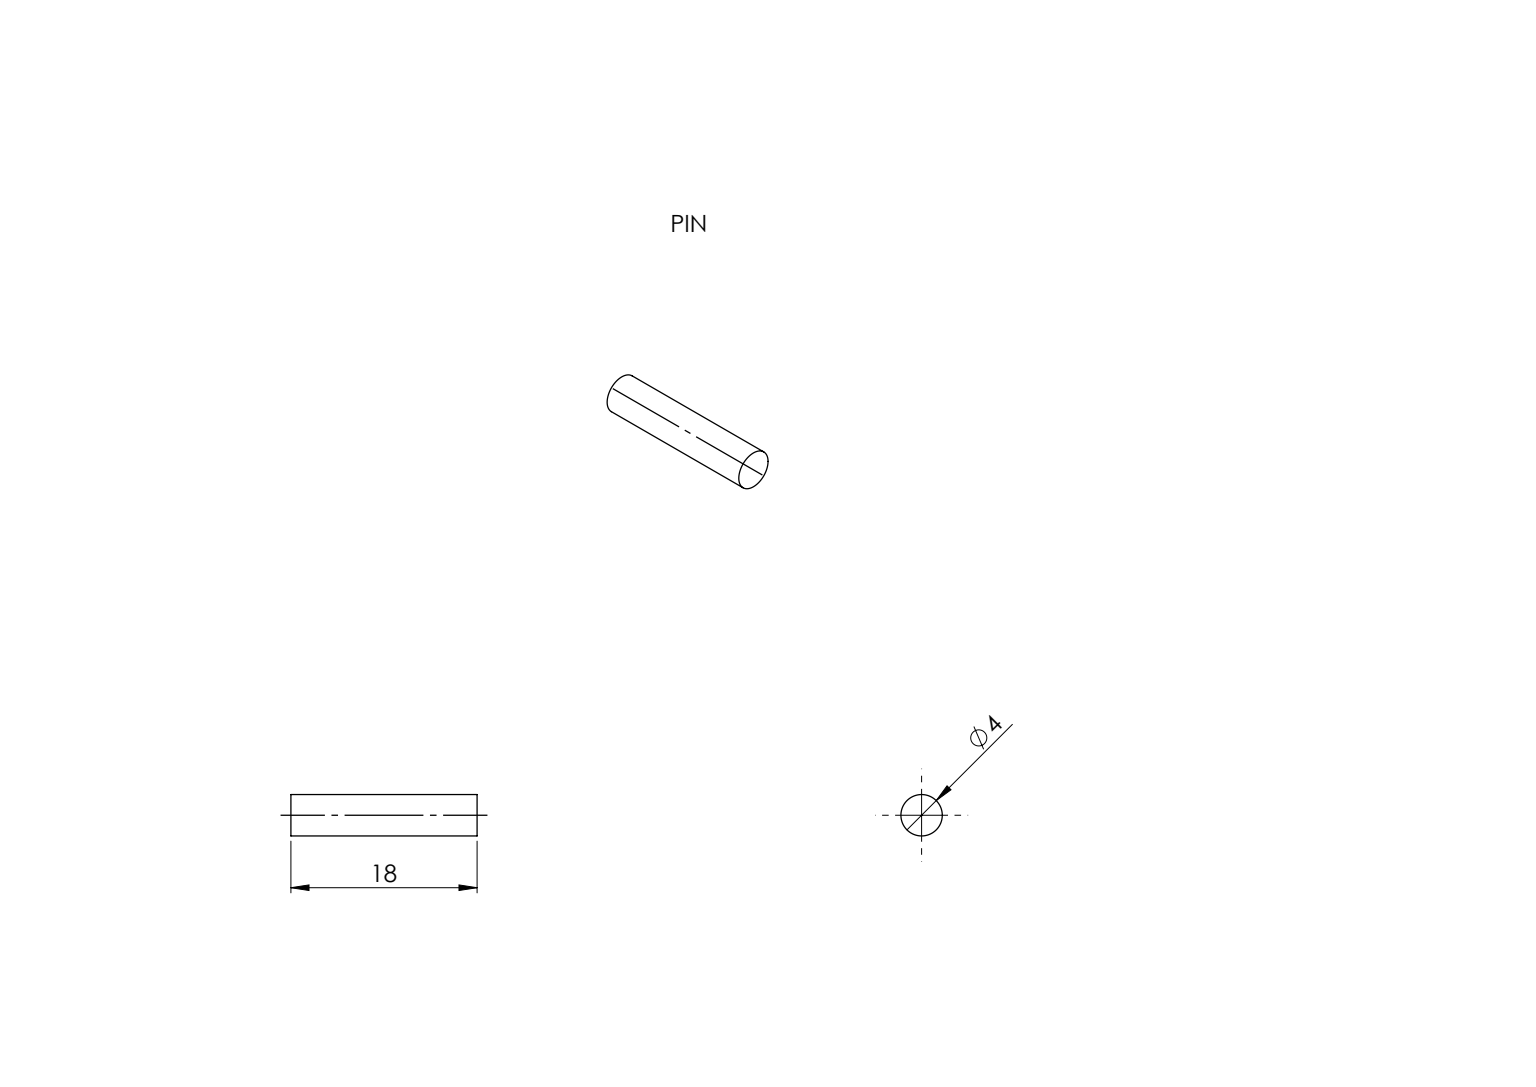
ISO-10303-21;
HEADER;
FILE_DESCRIPTION (('STEP AP214'),
    '1' );
FILE_NAME ('pin.step',
    '2026-10-03T18:28:46',
    ( '' ),
    ( '' ),
    'SwSTEP 2.0',
    'SolidWorks 2026',
    '' );
FILE_SCHEMA (( 'AUTOMOTIVE_DESIGN' ));
ENDSEC;

DATA;
#1=( LENGTH_UNIT ( ) NAMED_UNIT ( * ) SI_UNIT ( .MILLI., .METRE. ) );
#130=DIRECTION ( 'NONE',  ( 0.000000000000000000, 0.000000000000000000, -1.000000000000000000 ) ) ;
#220=ORIENTED_EDGE ( 'NONE', *, *, #9750, .F. ) ;
#239=CARTESIAN_POINT ( 'NONE',  ( 9.000000000000000000, 19.99999999999999645, 13.00000000000000000 ) ) ;
#291=DIRECTION ( 'NONE',  ( -1.000000000000000000, -0.000000000000000000, -0.000000000000000000 ) ) ;
#502=DIRECTION ( 'NONE',  ( 0.000000000000000000, 0.000000000000000000, 1.000000000000000000 ) ) ;
#644=SHAPE_DEFINITION_REPRESENTATION ( #7147, #9430 ) ;
#749=FACE_OUTER_BOUND ( 'NONE', #2071, .T. ) ;
#998=PRESENTATION_STYLE_ASSIGNMENT (( #4868 ) ) ;
#1023=ADVANCED_FACE ( 'NONE', ( #9629 ), #8663, .T. ) ;
#1105=ORIENTED_EDGE ( 'NONE', *, *, #3056, .F. ) ;
#1118=EDGE_CURVE ( 'NONE', #8741, #1470, #4721, .T. ) ;
#1207=ORIENTED_EDGE ( 'NONE', *, *, #4683, .F. ) ;
#1223=EDGE_CURVE ( 'NONE', #9435, #3589, #5730, .T. ) ;
#1293=DIRECTION ( 'NONE',  ( 1.000000000000000000, 0.000000000000000000, 0.000000000000000000 ) ) ;
#1299=CARTESIAN_POINT ( 'NONE',  ( 9.000000000000000000, 19.99999999999999645, 15.00000000000000000 ) ) ;
#1315=FACE_OUTER_BOUND ( 'NONE', #6062, .T. ) ;
#1470=VERTEX_POINT ( 'NONE', #5190 ) ;
#1784=( LENGTH_UNIT ( ) NAMED_UNIT ( * ) SI_UNIT ( .MILLI., .METRE. ) );
#2036=DIRECTION ( 'NONE',  ( 1.000000000000000000, 0.000000000000000000, 0.000000000000000000 ) ) ;
#2057=VECTOR ( 'NONE', #4305, 1000.000000000000000 ) ;
#2071=EDGE_LOOP ( 'NONE', ( #220, #10334, #2999, #7018 ) ) ;
#2090=DIRECTION ( 'NONE',  ( 0.000000000000000000, 0.000000000000000000, -1.000000000000000000 ) ) ;
#2101=AXIS2_PLACEMENT_3D ( 'NONE', #7090, #5610, #4547 ) ;
#2267=( GEOMETRIC_REPRESENTATION_CONTEXT ( 3 ) GLOBAL_UNCERTAINTY_ASSIGNED_CONTEXT ( ( #4377 ) ) GLOBAL_UNIT_ASSIGNED_CONTEXT ( ( #8113, #4925, #8273 ) ) REPRESENTATION_CONTEXT ( 'NONE', 'WORKASPACE' ) );
#2285=DIRECTION ( 'NONE',  ( -1.000000000000000000, -0.000000000000000000, -0.000000000000000000 ) ) ;
#2415=PRODUCT_DEFINITION_CONTEXT ( 'detailed design', #3097, 'design' ) ;
#2443=FILL_AREA_STYLE_COLOUR ( '', #7171 ) ;
#2493=FILL_AREA_STYLE ('',( #2443 ) ) ;
#2596=ADVANCED_FACE ( 'NONE', ( #8570 ), #2893, .T. ) ;
#2877=EDGE_CURVE ( 'NONE', #9435, #1470, #9790, .T. ) ;
#2893=CYLINDRICAL_SURFACE ( 'NONE', #5265, 2.000000000000001776 ) ;
#2947=( GEOMETRIC_REPRESENTATION_CONTEXT ( 3 ) GLOBAL_UNCERTAINTY_ASSIGNED_CONTEXT ( ( #3643 ) ) GLOBAL_UNIT_ASSIGNED_CONTEXT ( ( #1, #6456, #4125 ) ) REPRESENTATION_CONTEXT ( 'NONE', 'WORKASPACE' ) );
#2999=ORIENTED_EDGE ( 'NONE', *, *, #2877, .T. ) ;
#3056=EDGE_CURVE ( 'NONE', #3589, #9435, #8569, .T. ) ;
#3097=APPLICATION_CONTEXT ( 'automotive_design' ) ;
#3267=( NAMED_UNIT ( * ) PLANE_ANGLE_UNIT ( ) SI_UNIT ( $, .RADIAN. ) );
#3270=PRODUCT ( 'pin', 'pin', '', ( #8078 ) ) ;
#3440=ORIENTED_EDGE ( 'NONE', *, *, #2877, .F. ) ;
#3589=VERTEX_POINT ( 'NONE', #8495 ) ;
#3643=UNCERTAINTY_MEASURE_WITH_UNIT (LENGTH_MEASURE( 1.000000000000000082E-05 ), #1, 'distance_accuracy_value', 'NONE');
#3713=AXIS2_PLACEMENT_3D ( 'NONE', #4594, #5496, #7837 ) ;
#3716=ADVANCED_FACE ( 'NONE', ( #749 ), #8594, .T. ) ;
#3808=PRODUCT_DEFINITION_FORMATION_WITH_SPECIFIED_SOURCE ( 'ANY', '', #3270, .NOT_KNOWN. ) ;
#3845=FILL_AREA_STYLE_COLOUR ( '', #6596 ) ;
#4001=AXIS2_PLACEMENT_3D ( 'NONE', #9354, #2036, #2090 ) ;
#4125=( NAMED_UNIT ( * ) SI_UNIT ( $, .STERADIAN. ) SOLID_ANGLE_UNIT ( ) );
#4162=SURFACE_SIDE_STYLE ('',( #5742 ) ) ;
#4217=AXIS2_PLACEMENT_3D ( 'NONE', #6959, #1293, #4519 ) ;
#4305=DIRECTION ( 'NONE',  ( -1.000000000000000000, -0.000000000000000000, -0.000000000000000000 ) ) ;
#4349=ADVANCED_FACE ( 'NONE', ( #1315 ), #9491, .F. ) ;
#4374=ORIENTED_EDGE ( 'NONE', *, *, #1118, .F. ) ;
#4377=UNCERTAINTY_MEASURE_WITH_UNIT (LENGTH_MEASURE( 1.000000000000000082E-05 ), #8113, 'distance_accuracy_value', 'NONE');
#4416=CARTESIAN_POINT ( 'NONE',  ( -9.000000000000000000, 19.99999999999999645, 15.00000000000000000 ) ) ;
#4489=MANIFOLD_SOLID_BREP ( 'Boss-Extrude1', #6268 ) ;
#4519=DIRECTION ( 'NONE',  ( 0.000000000000000000, 0.000000000000000000, -1.000000000000000000 ) ) ;
#4547=DIRECTION ( 'NONE',  ( 1.000000000000000000, 0.000000000000000000, 0.000000000000000000 ) ) ;
#4594=CARTESIAN_POINT ( 'NONE',  ( -9.000000000000000000, 19.99999999999999645, 15.00000000000000000 ) ) ;
#4675=CARTESIAN_POINT ( 'NONE',  ( -9.000000000000000000, 19.99999999999999645, 13.00000000000000000 ) ) ;
#4683=EDGE_CURVE ( 'NONE', #1470, #8741, #6756, .T. ) ;
#4721=CIRCLE ( 'NONE', #4217, 2.000000000000000000 ) ;
#4868=SURFACE_STYLE_USAGE ( .BOTH. , #5705 ) ;
#4890=CARTESIAN_POINT ( 'NONE',  ( 9.000000000000000000, 19.99999999999999645, 15.00000000000000000 ) ) ;
#4906=( GEOMETRIC_REPRESENTATION_CONTEXT ( 3 ) GLOBAL_UNCERTAINTY_ASSIGNED_CONTEXT ( ( #8982 ) ) GLOBAL_UNIT_ASSIGNED_CONTEXT ( ( #1784, #3267, #7398 ) ) REPRESENTATION_CONTEXT ( 'NONE', 'WORKASPACE' ) );
#4925=( NAMED_UNIT ( * ) PLANE_ANGLE_UNIT ( ) SI_UNIT ( $, .RADIAN. ) );
#5162=DIRECTION ( 'NONE',  ( 0.000000000000000000, 0.000000000000000000, -1.000000000000000000 ) ) ;
#5190=CARTESIAN_POINT ( 'NONE',  ( -9.000000000000000000, 19.99999999999999645, 17.00000000000000000 ) ) ;
#5193=CARTESIAN_POINT ( 'NONE',  ( 9.000000000000000000, 19.99999999999999645, 17.00000000000000000 ) ) ;
#5265=AXIS2_PLACEMENT_3D ( 'NONE', #1299, #7770, #502 ) ;
#5496=DIRECTION ( 'NONE',  ( 1.000000000000000000, 0.000000000000000000, 0.000000000000000000 ) ) ;
#5509=DIRECTION ( 'NONE',  ( 0.000000000000000000, 0.000000000000000000, 1.000000000000000000 ) ) ;
#5579=STYLED_ITEM ( 'NONE', ( #5794 ), #4489 ) ;
#5610=DIRECTION ( 'NONE',  ( 0.000000000000000000, 0.000000000000000000, 1.000000000000000000 ) ) ;
#5705=SURFACE_SIDE_STYLE ('',( #8952 ) ) ;
#5730=CIRCLE ( 'NONE', #8152, 2.000000000000000000 ) ;
#5742=SURFACE_STYLE_FILL_AREA ( #10323 ) ;
#5794=PRESENTATION_STYLE_ASSIGNMENT (( #8837 ) ) ;
#5842=CARTESIAN_POINT ( 'NONE',  ( 9.000000000000000000, 19.99999999999999645, 17.00000000000000000 ) ) ;
#6062=EDGE_LOOP ( 'NONE', ( #1207, #4374 ) ) ;
#6123=PRODUCT_DEFINITION ( 'UNKNOWN', '', #3808, #2415 ) ;
#6268=CLOSED_SHELL ( 'NONE', ( #2596, #3716, #1023, #4349 ) ) ;
#6316=MECHANICAL_DESIGN_GEOMETRIC_PRESENTATION_REPRESENTATION('',(#7352),#2947);
#6431=ORIENTED_EDGE ( 'NONE', *, *, #1223, .T. ) ;
#6456=( NAMED_UNIT ( * ) PLANE_ANGLE_UNIT ( ) SI_UNIT ( $, .RADIAN. ) );
#6476=DIRECTION ( 'NONE',  ( 1.000000000000000000, 0.000000000000000000, 0.000000000000000000 ) ) ;
#6596=COLOUR_RGB ( '', 0.40784314, 0.44705882, 0.49803922) ;
#6756=CIRCLE ( 'NONE', #9312, 2.000000000000000000 ) ;
#6856=ORIENTED_EDGE ( 'NONE', *, *, #9750, .T. ) ;
#6884=APPLICATION_CONTEXT ( 'automotive_design' ) ;
#6959=CARTESIAN_POINT ( 'NONE',  ( -9.000000000000000000, 19.99999999999999645, 15.00000000000000000 ) ) ;
#7018=ORIENTED_EDGE ( 'NONE', *, *, #4683, .T. ) ;
#7090=CARTESIAN_POINT ( 'NONE',  ( 0.000000000000000000, 0.000000000000000000, 0.000000000000000000 ) ) ;
#7147=PRODUCT_DEFINITION_SHAPE ( 'NONE', 'NONE',  #6123 ) ;
#7171=COLOUR_RGB ( '', 0.40784314, 0.44705882, 0.49803922) ;
#7313=SHAPE_REPRESENTATION_RELATIONSHIP ( 'NONE' , 'NONE' ,  #9430, #9288 ) ;
#7352=STYLED_ITEM ( 'NONE', ( #998 ), #9288 ) ;
#7398=( NAMED_UNIT ( * ) SI_UNIT ( $, .STERADIAN. ) SOLID_ANGLE_UNIT ( ) );
#7616=MECHANICAL_DESIGN_GEOMETRIC_PRESENTATION_REPRESENTATION('',(#5579),#4906);
#7770=DIRECTION ( 'NONE',  ( -1.000000000000000000, -0.000000000000000000, -0.000000000000000000 ) ) ;
#7820=DIRECTION ( 'NONE',  ( 0.000000000000000000, 0.000000000000000000, -1.000000000000000000 ) ) ;
#7837=DIRECTION ( 'NONE',  ( 0.000000000000000000, 0.000000000000000000, -1.000000000000000000 ) ) ;
#7871=LINE ( 'NONE', #239, #9199 ) ;
#8078=PRODUCT_CONTEXT ( 'NONE', #6884, 'mechanical' ) ;
#8113=( LENGTH_UNIT ( ) NAMED_UNIT ( * ) SI_UNIT ( .MILLI., .METRE. ) );
#8152=AXIS2_PLACEMENT_3D ( 'NONE', #4890, #6476, #130 ) ;
#8273=( NAMED_UNIT ( * ) SI_UNIT ( $, .STERADIAN. ) SOLID_ANGLE_UNIT ( ) );
#8495=CARTESIAN_POINT ( 'NONE',  ( 9.000000000000000000, 19.99999999999999645, 13.00000000000000000 ) ) ;
#8508=ORIENTED_EDGE ( 'NONE', *, *, #1118, .T. ) ;
#8569=CIRCLE ( 'NONE', #4001, 2.000000000000000000 ) ;
#8570=FACE_OUTER_BOUND ( 'NONE', #9741, .T. ) ;
#8594=CYLINDRICAL_SURFACE ( 'NONE', #10271, 2.000000000000001776 ) ;
#8663=PLANE ( 'NONE',  #8796 ) ;
#8741=VERTEX_POINT ( 'NONE', #4675 ) ;
#8796=AXIS2_PLACEMENT_3D ( 'NONE', #9574, #9522, #7820 ) ;
#8837=SURFACE_STYLE_USAGE ( .BOTH. , #4162 ) ;
#8952=SURFACE_STYLE_FILL_AREA ( #2493 ) ;
#8982=UNCERTAINTY_MEASURE_WITH_UNIT (LENGTH_MEASURE( 1.000000000000000082E-05 ), #1784, 'distance_accuracy_value', 'NONE');
#9048=ORIENTED_EDGE ( 'NONE', *, *, #3056, .T. ) ;
#9118=EDGE_LOOP ( 'NONE', ( #6431, #9048 ) ) ;
#9199=VECTOR ( 'NONE', #291, 1000.000000000000000 ) ;
#9288=ADVANCED_BREP_SHAPE_REPRESENTATION ( '', ( #4489, #2101 ), #2267 ) ;
#9312=AXIS2_PLACEMENT_3D ( 'NONE', #4416, #9901, #5162 ) ;
#9354=CARTESIAN_POINT ( 'NONE',  ( 9.000000000000000000, 19.99999999999999645, 15.00000000000000000 ) ) ;
#9430=SHAPE_REPRESENTATION ( 'pin', ( #2101 ), #2267 ) ;
#9435=VERTEX_POINT ( 'NONE', #5193 ) ;
#9491=PLANE ( 'NONE',  #3713 ) ;
#9522=DIRECTION ( 'NONE',  ( 1.000000000000000000, 0.000000000000000000, 0.000000000000000000 ) ) ;
#9574=CARTESIAN_POINT ( 'NONE',  ( 9.000000000000000000, 19.99999999999999645, 15.00000000000000000 ) ) ;
#9629=FACE_OUTER_BOUND ( 'NONE', #9118, .T. ) ;
#9741=EDGE_LOOP ( 'NONE', ( #1105, #6856, #8508, #3440 ) ) ;
#9750=EDGE_CURVE ( 'NONE', #3589, #8741, #7871, .T. ) ;
#9790=LINE ( 'NONE', #5842, #2057 ) ;
#9901=DIRECTION ( 'NONE',  ( 1.000000000000000000, 0.000000000000000000, 0.000000000000000000 ) ) ;
#10271=AXIS2_PLACEMENT_3D ( 'NONE', #10297, #2285, #5509 ) ;
#10297=CARTESIAN_POINT ( 'NONE',  ( 9.000000000000000000, 19.99999999999999645, 15.00000000000000000 ) ) ;
#10323=FILL_AREA_STYLE ('',( #3845 ) ) ;
#10334=ORIENTED_EDGE ( 'NONE', *, *, #1223, .F. ) ;
ENDSEC;
END-ISO-10303-21;
